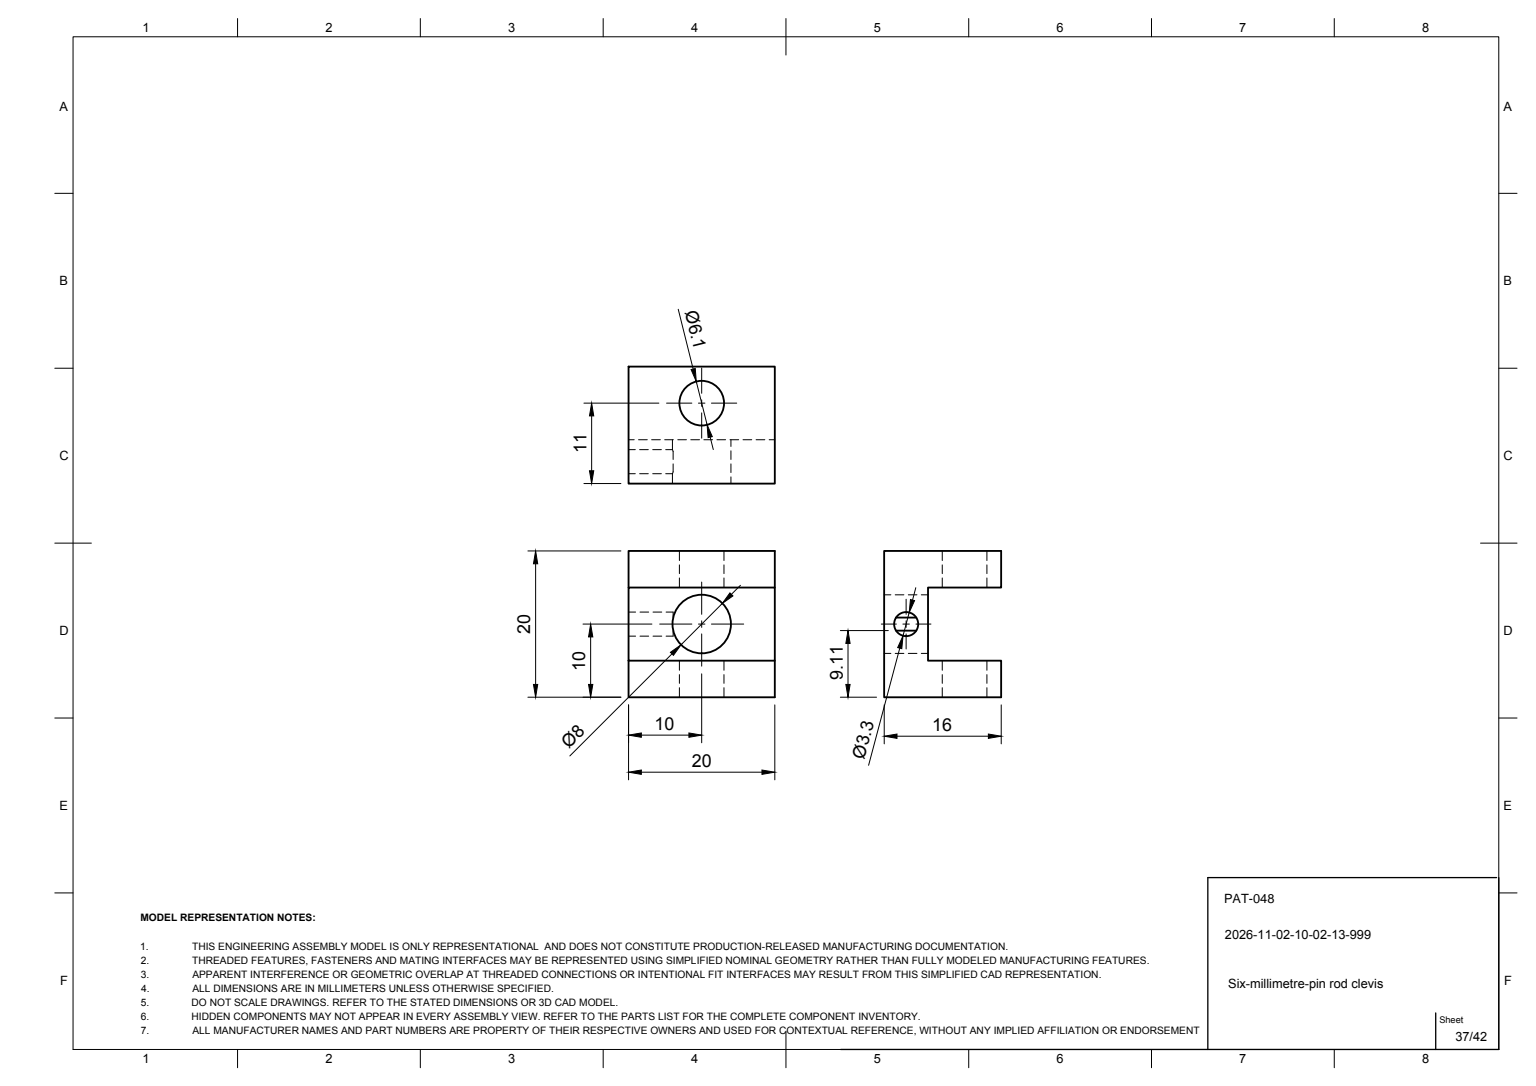
ISO-10303-21;
HEADER;
/* Generated by software containing ST-Developer
 * from STEP Tools, Inc. (www.steptools.com) 
 */

FILE_DESCRIPTION(
/* description */ ('Guided pneumatic stop gate'),
/* implementation_level */ '2;1');

FILE_NAME(
/* name */ 'Six-millimetre-pin rod clevis.step',
/* time_stamp */ '2026-10-27T21:43:45-07:00',
/* author */ (''),
/* organization */ (''),
/* preprocessor_version */ 'ST-DEVELOPER v20.2',
/* originating_system */ 'Autodesk Translation Framework v15.17.0.0',
/* authorisation */ '');

FILE_SCHEMA (('AUTOMOTIVE_DESIGN { 1 0 10303 214 3 1 1 }'));
ENDSEC;

DATA;
#10=MECHANICAL_DESIGN_GEOMETRIC_PRESENTATION_REPRESENTATION('',(#567),#14392);
#11=B_SPLINE_CURVE_WITH_KNOTS('',3,(#13750,#13751,#13752,#13753,#13754,
#13755,#13756,#13757,#13758,#13759),.UNSPECIFIED.,.F.,.F.,(4,2,2,2,4),(0.665271585430998,
0.692803751398643,0.75574615888762,0.818688566376597,0.846220732344242),
 .UNSPECIFIED.);
#12=B_SPLINE_CURVE_WITH_KNOTS('',3,(#13767,#13768,#13769,#13770,#13771,
#13772,#13773,#13774,#13775,#13776),.UNSPECIFIED.,.F.,.F.,(4,2,2,2,4),(0.161440812839251,
0.188972978806896,0.251915386295873,0.31485779378485,0.342389959752495),
 .UNSPECIFIED.);
#483=SHAPE_REPRESENTATION_RELATIONSHIP('SRR','None',#14620,#525);
#525=ADVANCED_BREP_SHAPE_REPRESENTATION('',(#605),#14382);
#567=STYLED_ITEM('',(#14891),#605);
#605=MANIFOLD_SOLID_BREP('Body1',#7911);
#798=FACE_BOUND('',#2173,.T.);
#799=FACE_BOUND('',#2175,.T.);
#800=FACE_BOUND('',#2177,.T.);
#801=FACE_BOUND('',#2179,.T.);
#802=FACE_BOUND('',#2184,.T.);
#803=FACE_BOUND('',#2186,.T.);
#804=FACE_BOUND('',#2188,.T.);
#805=FACE_BOUND('',#2190,.T.);
#1062=PLANE('',#9223);
#1063=PLANE('',#9229);
#1064=PLANE('',#9233);
#1065=PLANE('',#9234);
#1066=PLANE('',#9235);
#1067=PLANE('',#9236);
#1068=PLANE('',#9237);
#1069=PLANE('',#9238);
#1070=PLANE('',#9239);
#1071=PLANE('',#9240);
#1072=PLANE('',#9241);
#1073=PLANE('',#9242);
#1509=FACE_OUTER_BOUND('',#2167,.T.);
#1510=FACE_OUTER_BOUND('',#2168,.T.);
#1511=FACE_OUTER_BOUND('',#2169,.T.);
#1512=FACE_OUTER_BOUND('',#2170,.T.);
#1513=FACE_OUTER_BOUND('',#2171,.T.);
#1514=FACE_OUTER_BOUND('',#2172,.T.);
#1515=FACE_OUTER_BOUND('',#2174,.T.);
#1516=FACE_OUTER_BOUND('',#2176,.T.);
#1517=FACE_OUTER_BOUND('',#2178,.T.);
#1518=FACE_OUTER_BOUND('',#2180,.T.);
#1519=FACE_OUTER_BOUND('',#2181,.T.);
#1520=FACE_OUTER_BOUND('',#2182,.T.);
#1521=FACE_OUTER_BOUND('',#2183,.T.);
#1522=FACE_OUTER_BOUND('',#2185,.T.);
#1523=FACE_OUTER_BOUND('',#2187,.T.);
#1524=FACE_OUTER_BOUND('',#2189,.T.);
#2167=EDGE_LOOP('',(#6882,#6883,#6884,#6885));
#2168=EDGE_LOOP('',(#6886,#6887,#6888,#6889));
#2169=EDGE_LOOP('',(#6890,#6891));
#2170=EDGE_LOOP('',(#6892,#6893,#6894,#6895,#6896,#6897,#6898,#6899));
#2171=EDGE_LOOP('',(#6900,#6901,#6902));
#2172=EDGE_LOOP('',(#6903,#6904,#6905,#6906));
#2173=EDGE_LOOP('',(#6907,#6908,#6909,#6910));
#2174=EDGE_LOOP('',(#6911,#6912,#6913,#6914));
#2175=EDGE_LOOP('',(#6915));
#2176=EDGE_LOOP('',(#6916,#6917,#6918,#6919));
#2177=EDGE_LOOP('',(#6920));
#2178=EDGE_LOOP('',(#6921,#6922,#6923,#6924));
#2179=EDGE_LOOP('',(#6925));
#2180=EDGE_LOOP('',(#6926,#6927,#6928,#6929,#6930,#6931,#6932,#6933));
#2181=EDGE_LOOP('',(#6934,#6935,#6936,#6937));
#2182=EDGE_LOOP('',(#6938,#6939,#6940,#6941));
#2183=EDGE_LOOP('',(#6942,#6943,#6944,#6945));
#2184=EDGE_LOOP('',(#6946));
#2185=EDGE_LOOP('',(#6947,#6948,#6949,#6950));
#2186=EDGE_LOOP('',(#6951));
#2187=EDGE_LOOP('',(#6952,#6953,#6954,#6955));
#2188=EDGE_LOOP('',(#6956));
#2189=EDGE_LOOP('',(#6957,#6958,#6959,#6960,#6961,#6962,#6963,#6964));
#2190=EDGE_LOOP('',(#6965));
#2717=LINE('',#13735,#3262);
#2718=LINE('',#13741,#3263);
#2719=LINE('',#13746,#3264);
#2720=LINE('',#13763,#3265);
#2721=LINE('',#13778,#3266);
#2722=LINE('',#13783,#3267);
#2723=LINE('',#13788,#3268);
#2724=LINE('',#13790,#3269);
#2725=LINE('',#13792,#3270);
#2726=LINE('',#13793,#3271);
#2727=LINE('',#13796,#3272);
#2728=LINE('',#13798,#3273);
#2729=LINE('',#13799,#3274);
#2730=LINE('',#13802,#3275);
#2731=LINE('',#13804,#3276);
#2732=LINE('',#13805,#3277);
#2733=LINE('',#13808,#3278);
#2734=LINE('',#13810,#3279);
#2735=LINE('',#13812,#3280);
#2736=LINE('',#13814,#3281);
#2737=LINE('',#13815,#3282);
#2738=LINE('',#13818,#3283);
#2739=LINE('',#13819,#3284);
#2740=LINE('',#13822,#3285);
#2741=LINE('',#13823,#3286);
#2742=LINE('',#13826,#3287);
#2743=LINE('',#13828,#3288);
#2744=LINE('',#13829,#3289);
#2745=LINE('',#13831,#3290);
#2746=LINE('',#13833,#3291);
#3262=VECTOR('',#11490,0.305);
#3263=VECTOR('',#11497,0.305);
#3264=VECTOR('',#11502,1.);
#3265=VECTOR('',#11509,0.165);
#3266=VECTOR('',#11516,1.);
#3267=VECTOR('',#11521,0.4);
#3268=VECTOR('',#11526,1.);
#3269=VECTOR('',#11527,1.);
#3270=VECTOR('',#11528,1.);
#3271=VECTOR('',#11529,1.);
#3272=VECTOR('',#11532,1.);
#3273=VECTOR('',#11533,1.);
#3274=VECTOR('',#11534,1.);
#3275=VECTOR('',#11537,1.);
#3276=VECTOR('',#11538,1.);
#3277=VECTOR('',#11539,1.);
#3278=VECTOR('',#11542,1.);
#3279=VECTOR('',#11543,1.);
#3280=VECTOR('',#11544,1.);
#3281=VECTOR('',#11545,1.);
#3282=VECTOR('',#11546,1.);
#3283=VECTOR('',#11549,1.);
#3284=VECTOR('',#11550,1.);
#3285=VECTOR('',#11553,1.);
#3286=VECTOR('',#11554,1.);
#3287=VECTOR('',#11557,1.);
#3288=VECTOR('',#11558,1.);
#3289=VECTOR('',#11559,1.);
#3290=VECTOR('',#11562,1.);
#3291=VECTOR('',#11565,1.);
#3686=CIRCLE('',#9218,0.305);
#3687=CIRCLE('',#9219,0.305);
#3688=CIRCLE('',#9221,0.305);
#3689=CIRCLE('',#9222,0.305);
#3690=CIRCLE('',#9224,0.165);
#3691=CIRCLE('',#9226,0.165);
#3692=CIRCLE('',#9227,0.165);
#3693=CIRCLE('',#9228,0.165);
#3694=CIRCLE('',#9231,0.4);
#3695=CIRCLE('',#9232,0.4);
#4240=VERTEX_POINT('',#13732);
#4241=VERTEX_POINT('',#13734);
#4242=VERTEX_POINT('',#13738);
#4243=VERTEX_POINT('',#13740);
#4244=VERTEX_POINT('',#13744);
#4245=VERTEX_POINT('',#13745);
#4246=VERTEX_POINT('',#13749);
#4247=VERTEX_POINT('',#13760);
#4248=VERTEX_POINT('',#13762);
#4249=VERTEX_POINT('',#13765);
#4250=VERTEX_POINT('',#13780);
#4251=VERTEX_POINT('',#13782);
#4252=VERTEX_POINT('',#13786);
#4253=VERTEX_POINT('',#13787);
#4254=VERTEX_POINT('',#13789);
#4255=VERTEX_POINT('',#13791);
#4256=VERTEX_POINT('',#13795);
#4257=VERTEX_POINT('',#13797);
#4258=VERTEX_POINT('',#13801);
#4259=VERTEX_POINT('',#13803);
#4260=VERTEX_POINT('',#13807);
#4261=VERTEX_POINT('',#13809);
#4262=VERTEX_POINT('',#13811);
#4263=VERTEX_POINT('',#13813);
#4264=VERTEX_POINT('',#13817);
#4265=VERTEX_POINT('',#13821);
#4266=VERTEX_POINT('',#13825);
#4267=VERTEX_POINT('',#13827);
#5139=EDGE_CURVE('',#4240,#4240,#3686,.T.);
#5140=EDGE_CURVE('',#4240,#4241,#2717,.T.);
#5141=EDGE_CURVE('',#4241,#4241,#3687,.T.);
#5142=EDGE_CURVE('',#4242,#4242,#3688,.T.);
#5143=EDGE_CURVE('',#4242,#4243,#2718,.T.);
#5144=EDGE_CURVE('',#4243,#4243,#3689,.T.);
#5145=EDGE_CURVE('',#4244,#4245,#2719,.T.);
#5146=EDGE_CURVE('',#4244,#4245,#3690,.T.);
#5147=EDGE_CURVE('',#4246,#4244,#11,.T.);
#5148=EDGE_CURVE('',#4247,#4246,#3691,.T.);
#5149=EDGE_CURVE('',#4247,#4248,#2720,.T.);
#5150=EDGE_CURVE('',#4248,#4248,#3692,.T.);
#5151=EDGE_CURVE('',#4249,#4247,#3693,.T.);
#5152=EDGE_CURVE('',#4245,#4249,#12,.T.);
#5153=EDGE_CURVE('',#4249,#4246,#2721,.T.);
#5154=EDGE_CURVE('',#4250,#4250,#3694,.T.);
#5155=EDGE_CURVE('',#4250,#4251,#2722,.T.);
#5156=EDGE_CURVE('',#4251,#4251,#3695,.T.);
#5157=EDGE_CURVE('',#4252,#4253,#2723,.T.);
#5158=EDGE_CURVE('',#4254,#4252,#2724,.T.);
#5159=EDGE_CURVE('',#4255,#4254,#2725,.T.);
#5160=EDGE_CURVE('',#4253,#4255,#2726,.T.);
#5161=EDGE_CURVE('',#4256,#4252,#2727,.T.);
#5162=EDGE_CURVE('',#4257,#4256,#2728,.T.);
#5163=EDGE_CURVE('',#4254,#4257,#2729,.T.);
#5164=EDGE_CURVE('',#4258,#4256,#2730,.T.);
#5165=EDGE_CURVE('',#4259,#4258,#2731,.T.);
#5166=EDGE_CURVE('',#4257,#4259,#2732,.T.);
#5167=EDGE_CURVE('',#4260,#4259,#2733,.T.);
#5168=EDGE_CURVE('',#4261,#4260,#2734,.T.);
#5169=EDGE_CURVE('',#4262,#4261,#2735,.T.);
#5170=EDGE_CURVE('',#4263,#4262,#2736,.T.);
#5171=EDGE_CURVE('',#4255,#4263,#2737,.T.);
#5172=EDGE_CURVE('',#4264,#4258,#2738,.T.);
#5173=EDGE_CURVE('',#4260,#4264,#2739,.T.);
#5174=EDGE_CURVE('',#4263,#4265,#2740,.T.);
#5175=EDGE_CURVE('',#4253,#4265,#2741,.T.);
#5176=EDGE_CURVE('',#4261,#4266,#2742,.T.);
#5177=EDGE_CURVE('',#4267,#4266,#2743,.T.);
#5178=EDGE_CURVE('',#4262,#4267,#2744,.T.);
#5179=EDGE_CURVE('',#4265,#4267,#2745,.T.);
#5180=EDGE_CURVE('',#4266,#4264,#2746,.T.);
#6882=ORIENTED_EDGE('',*,*,#5139,.F.);
#6883=ORIENTED_EDGE('',*,*,#5140,.T.);
#6884=ORIENTED_EDGE('',*,*,#5141,.F.);
#6885=ORIENTED_EDGE('',*,*,#5140,.F.);
#6886=ORIENTED_EDGE('',*,*,#5142,.F.);
#6887=ORIENTED_EDGE('',*,*,#5143,.T.);
#6888=ORIENTED_EDGE('',*,*,#5144,.F.);
#6889=ORIENTED_EDGE('',*,*,#5143,.F.);
#6890=ORIENTED_EDGE('',*,*,#5145,.F.);
#6891=ORIENTED_EDGE('',*,*,#5146,.T.);
#6892=ORIENTED_EDGE('',*,*,#5147,.F.);
#6893=ORIENTED_EDGE('',*,*,#5148,.F.);
#6894=ORIENTED_EDGE('',*,*,#5149,.T.);
#6895=ORIENTED_EDGE('',*,*,#5150,.F.);
#6896=ORIENTED_EDGE('',*,*,#5149,.F.);
#6897=ORIENTED_EDGE('',*,*,#5151,.F.);
#6898=ORIENTED_EDGE('',*,*,#5152,.F.);
#6899=ORIENTED_EDGE('',*,*,#5146,.F.);
#6900=ORIENTED_EDGE('',*,*,#5153,.F.);
#6901=ORIENTED_EDGE('',*,*,#5151,.T.);
#6902=ORIENTED_EDGE('',*,*,#5148,.T.);
#6903=ORIENTED_EDGE('',*,*,#5154,.F.);
#6904=ORIENTED_EDGE('',*,*,#5155,.T.);
#6905=ORIENTED_EDGE('',*,*,#5156,.F.);
#6906=ORIENTED_EDGE('',*,*,#5155,.F.);
#6907=ORIENTED_EDGE('',*,*,#5152,.T.);
#6908=ORIENTED_EDGE('',*,*,#5153,.T.);
#6909=ORIENTED_EDGE('',*,*,#5147,.T.);
#6910=ORIENTED_EDGE('',*,*,#5145,.T.);
#6911=ORIENTED_EDGE('',*,*,#5157,.F.);
#6912=ORIENTED_EDGE('',*,*,#5158,.F.);
#6913=ORIENTED_EDGE('',*,*,#5159,.F.);
#6914=ORIENTED_EDGE('',*,*,#5160,.F.);
#6915=ORIENTED_EDGE('',*,*,#5142,.T.);
#6916=ORIENTED_EDGE('',*,*,#5161,.F.);
#6917=ORIENTED_EDGE('',*,*,#5162,.F.);
#6918=ORIENTED_EDGE('',*,*,#5163,.F.);
#6919=ORIENTED_EDGE('',*,*,#5158,.T.);
#6920=ORIENTED_EDGE('',*,*,#5154,.T.);
#6921=ORIENTED_EDGE('',*,*,#5164,.F.);
#6922=ORIENTED_EDGE('',*,*,#5165,.F.);
#6923=ORIENTED_EDGE('',*,*,#5166,.F.);
#6924=ORIENTED_EDGE('',*,*,#5162,.T.);
#6925=ORIENTED_EDGE('',*,*,#5141,.T.);
#6926=ORIENTED_EDGE('',*,*,#5159,.T.);
#6927=ORIENTED_EDGE('',*,*,#5163,.T.);
#6928=ORIENTED_EDGE('',*,*,#5166,.T.);
#6929=ORIENTED_EDGE('',*,*,#5167,.F.);
#6930=ORIENTED_EDGE('',*,*,#5168,.F.);
#6931=ORIENTED_EDGE('',*,*,#5169,.F.);
#6932=ORIENTED_EDGE('',*,*,#5170,.F.);
#6933=ORIENTED_EDGE('',*,*,#5171,.F.);
#6934=ORIENTED_EDGE('',*,*,#5165,.T.);
#6935=ORIENTED_EDGE('',*,*,#5172,.F.);
#6936=ORIENTED_EDGE('',*,*,#5173,.F.);
#6937=ORIENTED_EDGE('',*,*,#5167,.T.);
#6938=ORIENTED_EDGE('',*,*,#5160,.T.);
#6939=ORIENTED_EDGE('',*,*,#5171,.T.);
#6940=ORIENTED_EDGE('',*,*,#5174,.T.);
#6941=ORIENTED_EDGE('',*,*,#5175,.F.);
#6942=ORIENTED_EDGE('',*,*,#5169,.T.);
#6943=ORIENTED_EDGE('',*,*,#5176,.T.);
#6944=ORIENTED_EDGE('',*,*,#5177,.F.);
#6945=ORIENTED_EDGE('',*,*,#5178,.F.);
#6946=ORIENTED_EDGE('',*,*,#5156,.T.);
#6947=ORIENTED_EDGE('',*,*,#5170,.T.);
#6948=ORIENTED_EDGE('',*,*,#5178,.T.);
#6949=ORIENTED_EDGE('',*,*,#5179,.F.);
#6950=ORIENTED_EDGE('',*,*,#5174,.F.);
#6951=ORIENTED_EDGE('',*,*,#5144,.T.);
#6952=ORIENTED_EDGE('',*,*,#5168,.T.);
#6953=ORIENTED_EDGE('',*,*,#5173,.T.);
#6954=ORIENTED_EDGE('',*,*,#5180,.F.);
#6955=ORIENTED_EDGE('',*,*,#5176,.F.);
#6956=ORIENTED_EDGE('',*,*,#5139,.T.);
#6957=ORIENTED_EDGE('',*,*,#5157,.T.);
#6958=ORIENTED_EDGE('',*,*,#5175,.T.);
#6959=ORIENTED_EDGE('',*,*,#5179,.T.);
#6960=ORIENTED_EDGE('',*,*,#5177,.T.);
#6961=ORIENTED_EDGE('',*,*,#5180,.T.);
#6962=ORIENTED_EDGE('',*,*,#5172,.T.);
#6963=ORIENTED_EDGE('',*,*,#5164,.T.);
#6964=ORIENTED_EDGE('',*,*,#5161,.T.);
#6965=ORIENTED_EDGE('',*,*,#5150,.T.);
#7379=CYLINDRICAL_SURFACE('',#9217,0.305);
#7380=CYLINDRICAL_SURFACE('',#9220,0.305);
#7381=CYLINDRICAL_SURFACE('',#9225,0.165);
#7382=CYLINDRICAL_SURFACE('',#9230,0.4);
#7791=ADVANCED_FACE('',(#1509),#7379,.F.);
#7792=ADVANCED_FACE('',(#1510),#7380,.F.);
#7793=ADVANCED_FACE('',(#1511),#1062,.T.);
#7794=ADVANCED_FACE('',(#1512),#7381,.F.);
#7795=ADVANCED_FACE('',(#1513),#1063,.T.);
#7796=ADVANCED_FACE('',(#1514,#798),#7382,.F.);
#7797=ADVANCED_FACE('',(#1515,#799),#1064,.F.);
#7798=ADVANCED_FACE('',(#1516,#800),#1065,.F.);
#7799=ADVANCED_FACE('',(#1517,#801),#1066,.F.);
#7800=ADVANCED_FACE('',(#1518),#1067,.F.);
#7801=ADVANCED_FACE('',(#1519),#1068,.T.);
#7802=ADVANCED_FACE('',(#1520),#1069,.T.);
#7803=ADVANCED_FACE('',(#1521,#802),#1070,.T.);
#7804=ADVANCED_FACE('',(#1522,#803),#1071,.T.);
#7805=ADVANCED_FACE('',(#1523,#804),#1072,.T.);
#7806=ADVANCED_FACE('',(#1524,#805),#1073,.T.);
#7911=CLOSED_SHELL('',(#7791,#7792,#7793,#7794,#7795,#7796,#7797,#7798,
#7799,#7800,#7801,#7802,#7803,#7804,#7805,#7806));
#9216=AXIS2_PLACEMENT_3D('',#13730,#11484,#11485);
#9217=AXIS2_PLACEMENT_3D('',#13731,#11486,#11487);
#9218=AXIS2_PLACEMENT_3D('',#13733,#11488,#11489);
#9219=AXIS2_PLACEMENT_3D('',#13736,#11491,#11492);
#9220=AXIS2_PLACEMENT_3D('',#13737,#11493,#11494);
#9221=AXIS2_PLACEMENT_3D('',#13739,#11495,#11496);
#9222=AXIS2_PLACEMENT_3D('',#13742,#11498,#11499);
#9223=AXIS2_PLACEMENT_3D('',#13743,#11500,#11501);
#9224=AXIS2_PLACEMENT_3D('',#13747,#11503,#11504);
#9225=AXIS2_PLACEMENT_3D('',#13748,#11505,#11506);
#9226=AXIS2_PLACEMENT_3D('',#13761,#11507,#11508);
#9227=AXIS2_PLACEMENT_3D('',#13764,#11510,#11511);
#9228=AXIS2_PLACEMENT_3D('',#13766,#11512,#11513);
#9229=AXIS2_PLACEMENT_3D('',#13777,#11514,#11515);
#9230=AXIS2_PLACEMENT_3D('',#13779,#11517,#11518);
#9231=AXIS2_PLACEMENT_3D('',#13781,#11519,#11520);
#9232=AXIS2_PLACEMENT_3D('',#13784,#11522,#11523);
#9233=AXIS2_PLACEMENT_3D('',#13785,#11524,#11525);
#9234=AXIS2_PLACEMENT_3D('',#13794,#11530,#11531);
#9235=AXIS2_PLACEMENT_3D('',#13800,#11535,#11536);
#9236=AXIS2_PLACEMENT_3D('',#13806,#11540,#11541);
#9237=AXIS2_PLACEMENT_3D('',#13816,#11547,#11548);
#9238=AXIS2_PLACEMENT_3D('',#13820,#11551,#11552);
#9239=AXIS2_PLACEMENT_3D('',#13824,#11555,#11556);
#9240=AXIS2_PLACEMENT_3D('',#13830,#11560,#11561);
#9241=AXIS2_PLACEMENT_3D('',#13832,#11563,#11564);
#9242=AXIS2_PLACEMENT_3D('',#13834,#11566,#11567);
#11484=DIRECTION('axis',(0.,0.,1.));
#11485=DIRECTION('refdir',(1.,0.,0.));
#11486=DIRECTION('center_axis',(1.,0.,0.));
#11487=DIRECTION('ref_axis',(0.,0.,-1.));
#11488=DIRECTION('center_axis',(1.,0.,0.));
#11489=DIRECTION('ref_axis',(0.,0.,-1.));
#11490=DIRECTION('',(1.,0.,0.));
#11491=DIRECTION('center_axis',(-1.,0.,0.));
#11492=DIRECTION('ref_axis',(0.,0.,-1.));
#11493=DIRECTION('center_axis',(1.,0.,0.));
#11494=DIRECTION('ref_axis',(0.,0.,-1.));
#11495=DIRECTION('center_axis',(1.,0.,0.));
#11496=DIRECTION('ref_axis',(0.,0.,-1.));
#11497=DIRECTION('',(1.,0.,0.));
#11498=DIRECTION('center_axis',(-1.,0.,0.));
#11499=DIRECTION('ref_axis',(0.,0.,-1.));
#11500=DIRECTION('center_axis',(0.,0.,1.));
#11501=DIRECTION('ref_axis',(1.,0.,0.));
#11502=DIRECTION('',(0.,1.,0.));
#11503=DIRECTION('center_axis',(0.,0.,1.));
#11504=DIRECTION('ref_axis',(1.,0.,0.));
#11505=DIRECTION('center_axis',(0.,0.,1.));
#11506=DIRECTION('ref_axis',(1.,0.,0.));
#11507=DIRECTION('center_axis',(0.,0.,1.));
#11508=DIRECTION('ref_axis',(1.,0.,0.));
#11509=DIRECTION('',(0.,0.,1.));
#11510=DIRECTION('center_axis',(0.,0.,-1.));
#11511=DIRECTION('ref_axis',(1.,0.,0.));
#11512=DIRECTION('center_axis',(0.,0.,1.));
#11513=DIRECTION('ref_axis',(1.,0.,0.));
#11514=DIRECTION('center_axis',(0.,0.,1.));
#11515=DIRECTION('ref_axis',(1.,0.,0.));
#11516=DIRECTION('',(0.,-1.,0.));
#11517=DIRECTION('center_axis',(0.,1.,0.));
#11518=DIRECTION('ref_axis',(1.,0.,0.));
#11519=DIRECTION('center_axis',(0.,1.,0.));
#11520=DIRECTION('ref_axis',(1.,0.,0.));
#11521=DIRECTION('',(0.,1.,0.));
#11522=DIRECTION('center_axis',(0.,-1.,0.));
#11523=DIRECTION('ref_axis',(1.,0.,0.));
#11524=DIRECTION('center_axis',(1.,0.,0.));
#11525=DIRECTION('ref_axis',(0.,1.,0.));
#11526=DIRECTION('',(0.,-1.,0.));
#11527=DIRECTION('',(0.,0.,1.));
#11528=DIRECTION('',(0.,1.,0.));
#11529=DIRECTION('',(0.,0.,-1.));
#11530=DIRECTION('center_axis',(0.,1.,0.));
#11531=DIRECTION('ref_axis',(-1.,0.,0.));
#11532=DIRECTION('',(1.,0.,0.));
#11533=DIRECTION('',(0.,0.,1.));
#11534=DIRECTION('',(-1.,0.,0.));
#11535=DIRECTION('center_axis',(-1.,0.,0.));
#11536=DIRECTION('ref_axis',(0.,-1.,0.));
#11537=DIRECTION('',(0.,1.,0.));
#11538=DIRECTION('',(0.,0.,1.));
#11539=DIRECTION('',(0.,-1.,0.));
#11540=DIRECTION('center_axis',(0.,0.,1.));
#11541=DIRECTION('ref_axis',(1.,0.,0.));
#11542=DIRECTION('',(1.,0.,0.));
#11543=DIRECTION('',(0.,-1.,0.));
#11544=DIRECTION('',(-1.,0.,0.));
#11545=DIRECTION('',(0.,1.,0.));
#11546=DIRECTION('',(1.,0.,0.));
#11547=DIRECTION('center_axis',(0.,-1.,0.));
#11548=DIRECTION('ref_axis',(1.,0.,0.));
#11549=DIRECTION('',(1.,0.,0.));
#11550=DIRECTION('',(0.,0.,1.));
#11551=DIRECTION('center_axis',(0.,-1.,0.));
#11552=DIRECTION('ref_axis',(1.,0.,0.));
#11553=DIRECTION('',(0.,0.,1.));
#11554=DIRECTION('',(1.,0.,0.));
#11555=DIRECTION('center_axis',(0.,1.,0.));
#11556=DIRECTION('ref_axis',(-1.,0.,0.));
#11557=DIRECTION('',(0.,0.,1.));
#11558=DIRECTION('',(-1.,0.,0.));
#11559=DIRECTION('',(0.,0.,1.));
#11560=DIRECTION('center_axis',(1.,0.,0.));
#11561=DIRECTION('ref_axis',(0.,1.,0.));
#11562=DIRECTION('',(0.,1.,0.));
#11563=DIRECTION('center_axis',(-1.,0.,0.));
#11564=DIRECTION('ref_axis',(0.,-1.,0.));
#11565=DIRECTION('',(0.,-1.,0.));
#11566=DIRECTION('center_axis',(0.,0.,1.));
#11567=DIRECTION('ref_axis',(1.,0.,0.));
#13730=CARTESIAN_POINT('',(0.,0.,0.));
#13731=CARTESIAN_POINT('Origin',(-1.1,-6.1,4.5));
#13732=CARTESIAN_POINT('',(-1.,-6.1,4.805));
#13733=CARTESIAN_POINT('Origin',(-1.,-6.1,4.5));
#13734=CARTESIAN_POINT('',(-0.5,-6.1,4.805));
#13735=CARTESIAN_POINT('',(-1.1,-6.1,4.805));
#13736=CARTESIAN_POINT('Origin',(-0.5,-6.1,4.5));
#13737=CARTESIAN_POINT('Origin',(-1.1,-6.1,4.5));
#13738=CARTESIAN_POINT('',(0.5,-6.1,4.805));
#13739=CARTESIAN_POINT('Origin',(0.5,-6.1,4.5));
#13740=CARTESIAN_POINT('',(1.,-6.1,4.805));
#13741=CARTESIAN_POINT('',(-1.1,-6.1,4.805));
#13742=CARTESIAN_POINT('Origin',(1.,-6.1,4.5));
#13743=CARTESIAN_POINT('Origin',(0.,-5.3,4.89));
#13744=CARTESIAN_POINT('',(0.0888819441731535,-5.43901438774458,4.89));
#13745=CARTESIAN_POINT('',(0.0888819441731535,-5.16098561225542,4.89));
#13746=CARTESIAN_POINT('',(0.0888819441731535,-5.6,4.89));
#13747=CARTESIAN_POINT('Origin',(0.,-5.3,4.89));
#13748=CARTESIAN_POINT('Origin',(0.,-5.3,4.89));
#13749=CARTESIAN_POINT('',(-0.0888819441731535,-5.43901438774458,4.89));
#13750=CARTESIAN_POINT('Ctrl Pts',(-0.0888819441731541,-5.43901438774458,
4.89));
#13751=CARTESIAN_POINT('Ctrl Pts',(-0.0808964434200148,-5.44412009546053,
4.89181991495419));
#13752=CARTESIAN_POINT('Ctrl Pts',(-0.0723643333023662,-5.44859639186021,
4.89350251788328));
#13753=CARTESIAN_POINT('Ctrl Pts',(-0.0431949313468613,-5.46075622416973,
4.89819171553211));
#13754=CARTESIAN_POINT('Ctrl Pts',(-0.0209808024963256,-5.465,4.9));
#13755=CARTESIAN_POINT('Ctrl Pts',(0.0209808024963256,-5.465,4.9));
#13756=CARTESIAN_POINT('Ctrl Pts',(0.0431949313468613,-5.46075622416973,
4.89819171553211));
#13757=CARTESIAN_POINT('Ctrl Pts',(0.0723643333023662,-5.44859639186021,
4.89350251788328));
#13758=CARTESIAN_POINT('Ctrl Pts',(0.0808964434200144,-5.44412009546053,
4.89181991495419));
#13759=CARTESIAN_POINT('Ctrl Pts',(0.0888819441731541,-5.43901438774458,
4.89));
#13760=CARTESIAN_POINT('',(-0.165,-5.3,4.89));
#13761=CARTESIAN_POINT('Origin',(0.,-5.3,4.89));
#13762=CARTESIAN_POINT('',(-0.165,-5.3,5.5));
#13763=CARTESIAN_POINT('',(-0.165,-5.3,4.89));
#13764=CARTESIAN_POINT('Origin',(0.,-5.3,5.5));
#13765=CARTESIAN_POINT('',(-0.0888819441731535,-5.16098561225542,4.89));
#13766=CARTESIAN_POINT('Origin',(0.,-5.3,4.89));
#13767=CARTESIAN_POINT('Ctrl Pts',(0.0888819441731536,-5.16098561225542,
4.89));
#13768=CARTESIAN_POINT('Ctrl Pts',(0.0808964434200141,-5.15587990453947,
4.89181991495419));
#13769=CARTESIAN_POINT('Ctrl Pts',(0.0723643333023662,-5.15140360813979,
4.89350251788328));
#13770=CARTESIAN_POINT('Ctrl Pts',(0.0431949313468613,-5.13924377583027,
4.89819171553211));
#13771=CARTESIAN_POINT('Ctrl Pts',(0.0209808024963256,-5.135,4.9));
#13772=CARTESIAN_POINT('Ctrl Pts',(-0.0209808024963256,-5.135,4.9));
#13773=CARTESIAN_POINT('Ctrl Pts',(-0.0431949313468613,-5.13924377583027,
4.89819171553211));
#13774=CARTESIAN_POINT('Ctrl Pts',(-0.0723643333023663,-5.15140360813979,
4.89350251788328));
#13775=CARTESIAN_POINT('Ctrl Pts',(-0.0808964434200144,-5.15587990453947,
4.89181991495419));
#13776=CARTESIAN_POINT('Ctrl Pts',(-0.0888819441731536,-5.16098561225542,
4.89));
#13777=CARTESIAN_POINT('Origin',(0.,-5.3,4.89));
#13778=CARTESIAN_POINT('',(-0.0888819441731535,-5.6,4.89));
#13779=CARTESIAN_POINT('Origin',(0.,-5.6,4.5));
#13780=CARTESIAN_POINT('',(-0.4,-5.6,4.5));
#13781=CARTESIAN_POINT('Origin',(0.,-5.6,4.5));
#13782=CARTESIAN_POINT('',(-0.4,-5.,4.5));
#13783=CARTESIAN_POINT('',(-0.4,-5.6,4.5));
#13784=CARTESIAN_POINT('Origin',(0.,-5.,4.5));
#13785=CARTESIAN_POINT('Origin',(0.5,-6.7,3.4));
#13786=CARTESIAN_POINT('',(0.5,-5.6,5.5));
#13787=CARTESIAN_POINT('',(0.5,-6.6,5.5));
#13788=CARTESIAN_POINT('',(0.5,-6.25,5.5));
#13789=CARTESIAN_POINT('',(0.5,-5.6,3.5));
#13790=CARTESIAN_POINT('',(0.5,-5.6,3.4));
#13791=CARTESIAN_POINT('',(0.5,-6.6,3.5));
#13792=CARTESIAN_POINT('',(0.5,-6.25,3.5));
#13793=CARTESIAN_POINT('',(0.5,-6.6,3.45));
#13794=CARTESIAN_POINT('Origin',(0.5,-5.6,3.4));
#13795=CARTESIAN_POINT('',(-0.5,-5.6,5.5));
#13796=CARTESIAN_POINT('',(0.25,-5.6,5.5));
#13797=CARTESIAN_POINT('',(-0.5,-5.6,3.5));
#13798=CARTESIAN_POINT('',(-0.5,-5.6,3.4));
#13799=CARTESIAN_POINT('',(0.25,-5.6,3.5));
#13800=CARTESIAN_POINT('Origin',(-0.5,-5.6,3.4));
#13801=CARTESIAN_POINT('',(-0.5,-6.6,5.5));
#13802=CARTESIAN_POINT('',(-0.5,-5.7,5.5));
#13803=CARTESIAN_POINT('',(-0.5,-6.6,3.5));
#13804=CARTESIAN_POINT('',(-0.5,-6.6,3.45));
#13805=CARTESIAN_POINT('',(-0.5,-5.7,3.5));
#13806=CARTESIAN_POINT('Origin',(0.,-5.8,3.5));
#13807=CARTESIAN_POINT('',(-1.,-6.6,3.5));
#13808=CARTESIAN_POINT('',(-1.,-6.6,3.5));
#13809=CARTESIAN_POINT('',(-1.,-5.,3.5));
#13810=CARTESIAN_POINT('',(-1.,-5.,3.5));
#13811=CARTESIAN_POINT('',(1.,-5.,3.5));
#13812=CARTESIAN_POINT('',(1.,-5.,3.5));
#13813=CARTESIAN_POINT('',(1.,-6.6,3.5));
#13814=CARTESIAN_POINT('',(1.,-6.6,3.5));
#13815=CARTESIAN_POINT('',(-1.,-6.6,3.5));
#13816=CARTESIAN_POINT('Origin',(-1.,-6.6,3.5));
#13817=CARTESIAN_POINT('',(-1.,-6.6,5.5));
#13818=CARTESIAN_POINT('',(-1.,-6.6,5.5));
#13819=CARTESIAN_POINT('',(-1.,-6.6,3.5));
#13820=CARTESIAN_POINT('Origin',(-1.,-6.6,3.5));
#13821=CARTESIAN_POINT('',(1.,-6.6,5.5));
#13822=CARTESIAN_POINT('',(1.,-6.6,3.5));
#13823=CARTESIAN_POINT('',(-1.,-6.6,5.5));
#13824=CARTESIAN_POINT('Origin',(1.,-5.,3.5));
#13825=CARTESIAN_POINT('',(-1.,-5.,5.5));
#13826=CARTESIAN_POINT('',(-1.,-5.,3.5));
#13827=CARTESIAN_POINT('',(1.,-5.,5.5));
#13828=CARTESIAN_POINT('',(1.,-5.,5.5));
#13829=CARTESIAN_POINT('',(1.,-5.,3.5));
#13830=CARTESIAN_POINT('Origin',(1.,-6.6,3.5));
#13831=CARTESIAN_POINT('',(1.,-6.6,5.5));
#13832=CARTESIAN_POINT('Origin',(-1.,-5.,3.5));
#13833=CARTESIAN_POINT('',(-1.,-5.,5.5));
#13834=CARTESIAN_POINT('Origin',(0.,-5.8,5.5));
#14334=UNCERTAINTY_MEASURE_WITH_UNIT(LENGTH_MEASURE(0.001),#14393,
'DISTANCE_ACCURACY_VALUE',
'Maximum model space distance between geometric entities at asserted c
onnectivities');
#14344=UNCERTAINTY_MEASURE_WITH_UNIT(LENGTH_MEASURE(0.001),#14393,
'DISTANCE_ACCURACY_VALUE',
'Maximum model space distance between geometric entities at asserted c
onnectivities');
#14382=(
GEOMETRIC_REPRESENTATION_CONTEXT(3)
GLOBAL_UNCERTAINTY_ASSIGNED_CONTEXT((#14334))
GLOBAL_UNIT_ASSIGNED_CONTEXT((#14393,#14395,#14396))
REPRESENTATION_CONTEXT('','3D')
);
#14392=(
GEOMETRIC_REPRESENTATION_CONTEXT(3)
GLOBAL_UNCERTAINTY_ASSIGNED_CONTEXT((#14344))
GLOBAL_UNIT_ASSIGNED_CONTEXT((#14393,#14395,#14396))
REPRESENTATION_CONTEXT('','3D')
);
#14393=(
LENGTH_UNIT()
NAMED_UNIT(*)
SI_UNIT(.CENTI.,.METRE.)
);
#14395=(
NAMED_UNIT(*)
PLANE_ANGLE_UNIT()
SI_UNIT($,.RADIAN.)
);
#14396=(
NAMED_UNIT(*)
SI_UNIT($,.STERADIAN.)
SOLID_ANGLE_UNIT()
);
#14434=SHAPE_DEFINITION_REPRESENTATION(#14553,#14620);
#14553=PRODUCT_DEFINITION_SHAPE('',$,#14668);
#14620=SHAPE_REPRESENTATION('',(#9216),#14382);
#14630=PRODUCT_DEFINITION_CONTEXT('part definition',#14773,'design');
#14668=PRODUCT_DEFINITION('Six-millimetre-pin rod clevis',
'Six-millimetre-pin rod clevis',#14715,#14630);
#14715=PRODUCT_DEFINITION_FORMATION('',$,#14812);
#14773=APPLICATION_CONTEXT(
'Core Data for Automotive Mechanical Design Process');
#14774=PRODUCT_CONTEXT('part definition',#14773,'mechanical');
#14812=PRODUCT('Six-millimetre-pin rod clevis',
'Six-millimetre-pin rod clevis','Six-millimetre-pin rod clevis',(#14774));
#14885=COLOUR_RGB('Grey',0.48,0.52,0.57);
#14886=FILL_AREA_STYLE_COLOUR('',#14885);
#14887=FILL_AREA_STYLE('',(#14886));
#14888=SURFACE_STYLE_FILL_AREA(#14887);
#14889=SURFACE_SIDE_STYLE('',(#14888));
#14890=SURFACE_STYLE_USAGE(.BOTH.,#14889);
#14891=PRESENTATION_STYLE_ASSIGNMENT((#14890));
ENDSEC;
END-ISO-10303-21;
